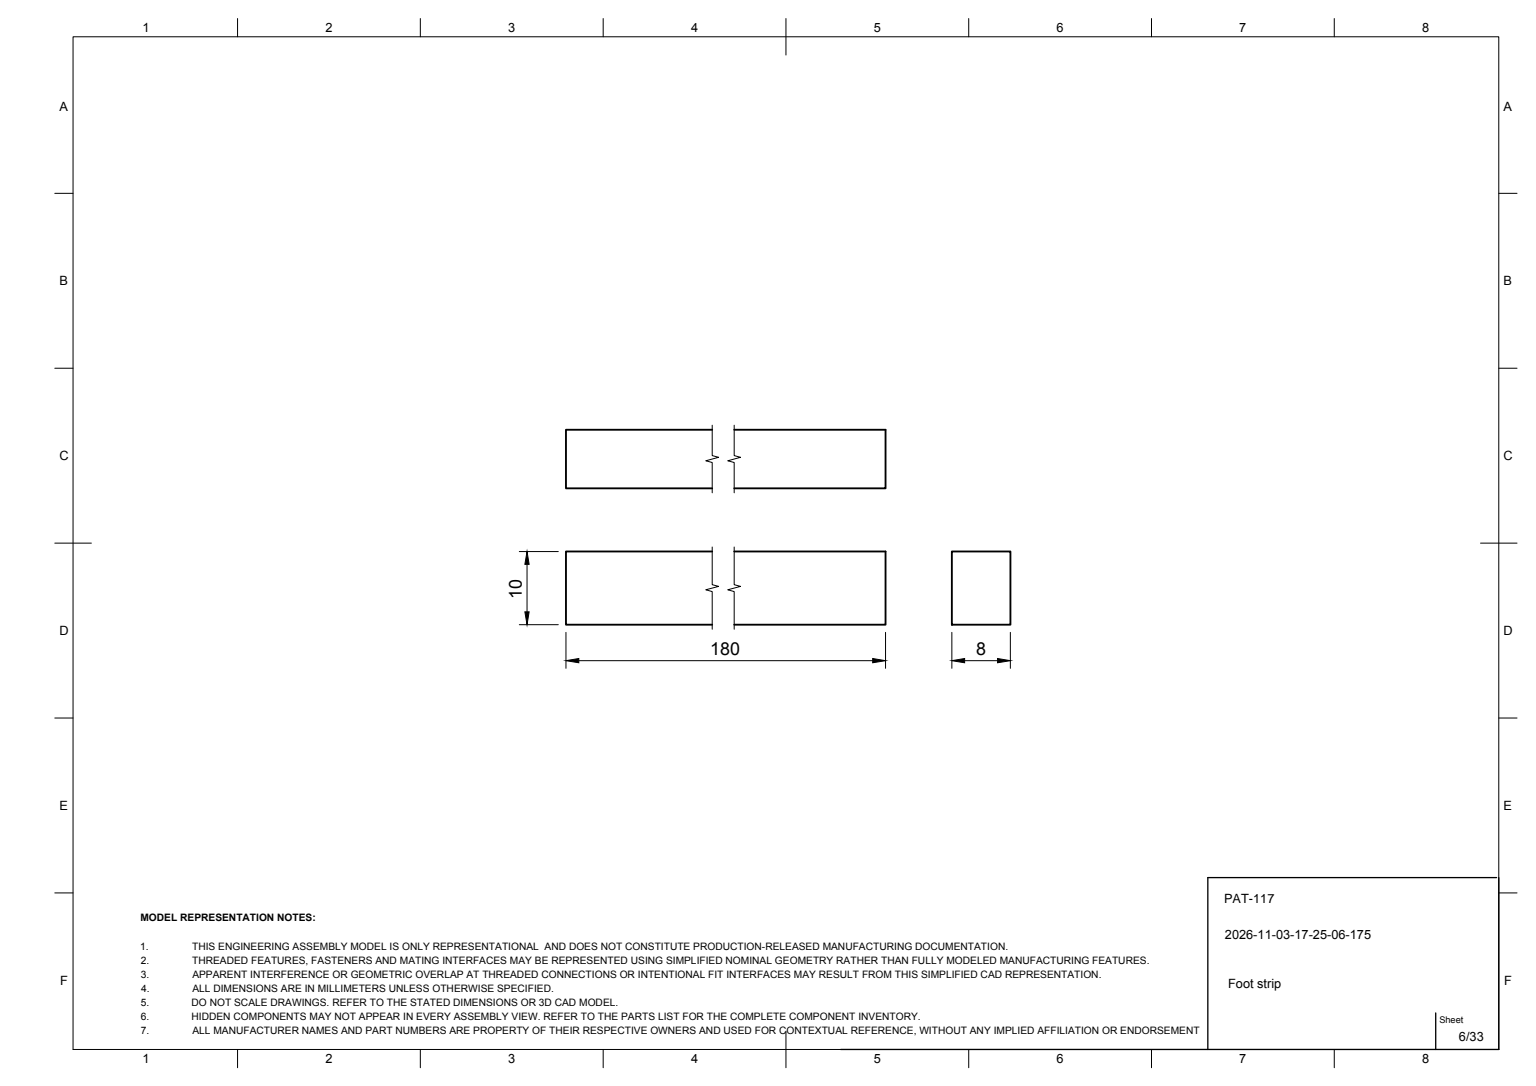
ISO-10303-21;
HEADER;
/* Generated by software containing ST-Developer
 * from STEP Tools, Inc. (www.steptools.com) 
 */

FILE_DESCRIPTION(
/* description */ ('Counterbalanced vertical column'),
/* implementation_level */ '2;1');

FILE_NAME(
/* name */ 'Foot strip.step',
/* time_stamp */ '2026-10-29T16:47:22-07:00',
/* author */ (''),
/* organization */ (''),
/* preprocessor_version */ 'ST-DEVELOPER v20.2',
/* originating_system */ 'Autodesk Translation Framework v15.17.0.0',
/* authorisation */ '');

FILE_SCHEMA (('AUTOMOTIVE_DESIGN { 1 0 10303 214 3 1 1 }'));
ENDSEC;

DATA;
#10=MECHANICAL_DESIGN_GEOMETRIC_PRESENTATION_REPRESENTATION('',(#351),#15040);
#281=SHAPE_REPRESENTATION_RELATIONSHIP('SRR','None',#15185,#316);
#316=ADVANCED_BREP_SHAPE_REPRESENTATION('',(#386),#15004);
#351=STYLED_ITEM('',(#15443),#386);
#386=MANIFOLD_SOLID_BREP('Body1',#7074);
#541=PLANE('',#7527);
#542=PLANE('',#7528);
#543=PLANE('',#7529);
#544=PLANE('',#7530);
#545=PLANE('',#7531);
#546=PLANE('',#7532);
#841=FACE_OUTER_BOUND('',#1252,.T.);
#842=FACE_OUTER_BOUND('',#1253,.T.);
#843=FACE_OUTER_BOUND('',#1254,.T.);
#844=FACE_OUTER_BOUND('',#1255,.T.);
#845=FACE_OUTER_BOUND('',#1256,.T.);
#846=FACE_OUTER_BOUND('',#1257,.T.);
#1252=EDGE_LOOP('',(#4842,#4843,#4844,#4845));
#1253=EDGE_LOOP('',(#4846,#4847,#4848,#4849));
#1254=EDGE_LOOP('',(#4850,#4851,#4852,#4853));
#1255=EDGE_LOOP('',(#4854,#4855,#4856,#4857));
#1256=EDGE_LOOP('',(#4858,#4859,#4860,#4861));
#1257=EDGE_LOOP('',(#4862,#4863,#4864,#4865));
#1768=LINE('',#10405,#2439);
#1769=LINE('',#10407,#2440);
#1770=LINE('',#10409,#2441);
#1771=LINE('',#10410,#2442);
#1772=LINE('',#10413,#2443);
#1773=LINE('',#10415,#2444);
#1774=LINE('',#10416,#2445);
#1775=LINE('',#10419,#2446);
#1776=LINE('',#10421,#2447);
#1777=LINE('',#10422,#2448);
#1778=LINE('',#10424,#2449);
#1779=LINE('',#10425,#2450);
#2439=VECTOR('',#8298,1.);
#2440=VECTOR('',#8299,1.);
#2441=VECTOR('',#8300,1.);
#2442=VECTOR('',#8301,1.);
#2443=VECTOR('',#8304,1.);
#2444=VECTOR('',#8305,1.);
#2445=VECTOR('',#8306,1.);
#2446=VECTOR('',#8309,1.);
#2447=VECTOR('',#8310,1.);
#2448=VECTOR('',#8311,1.);
#2449=VECTOR('',#8314,1.);
#2450=VECTOR('',#8315,1.);
#3324=VERTEX_POINT('',#10403);
#3325=VERTEX_POINT('',#10404);
#3326=VERTEX_POINT('',#10406);
#3327=VERTEX_POINT('',#10408);
#3328=VERTEX_POINT('',#10412);
#3329=VERTEX_POINT('',#10414);
#3330=VERTEX_POINT('',#10418);
#3331=VERTEX_POINT('',#10420);
#3922=EDGE_CURVE('',#3324,#3325,#1768,.T.);
#3923=EDGE_CURVE('',#3325,#3326,#1769,.T.);
#3924=EDGE_CURVE('',#3327,#3326,#1770,.T.);
#3925=EDGE_CURVE('',#3324,#3327,#1771,.T.);
#3926=EDGE_CURVE('',#3328,#3324,#1772,.T.);
#3927=EDGE_CURVE('',#3329,#3327,#1773,.T.);
#3928=EDGE_CURVE('',#3328,#3329,#1774,.T.);
#3929=EDGE_CURVE('',#3330,#3328,#1775,.T.);
#3930=EDGE_CURVE('',#3331,#3329,#1776,.T.);
#3931=EDGE_CURVE('',#3330,#3331,#1777,.T.);
#3932=EDGE_CURVE('',#3325,#3330,#1778,.T.);
#3933=EDGE_CURVE('',#3326,#3331,#1779,.T.);
#4842=ORIENTED_EDGE('',*,*,#3922,.T.);
#4843=ORIENTED_EDGE('',*,*,#3923,.T.);
#4844=ORIENTED_EDGE('',*,*,#3924,.F.);
#4845=ORIENTED_EDGE('',*,*,#3925,.F.);
#4846=ORIENTED_EDGE('',*,*,#3926,.T.);
#4847=ORIENTED_EDGE('',*,*,#3925,.T.);
#4848=ORIENTED_EDGE('',*,*,#3927,.F.);
#4849=ORIENTED_EDGE('',*,*,#3928,.F.);
#4850=ORIENTED_EDGE('',*,*,#3929,.T.);
#4851=ORIENTED_EDGE('',*,*,#3928,.T.);
#4852=ORIENTED_EDGE('',*,*,#3930,.F.);
#4853=ORIENTED_EDGE('',*,*,#3931,.F.);
#4854=ORIENTED_EDGE('',*,*,#3932,.T.);
#4855=ORIENTED_EDGE('',*,*,#3931,.T.);
#4856=ORIENTED_EDGE('',*,*,#3933,.F.);
#4857=ORIENTED_EDGE('',*,*,#3923,.F.);
#4858=ORIENTED_EDGE('',*,*,#3933,.T.);
#4859=ORIENTED_EDGE('',*,*,#3930,.T.);
#4860=ORIENTED_EDGE('',*,*,#3927,.T.);
#4861=ORIENTED_EDGE('',*,*,#3924,.T.);
#4862=ORIENTED_EDGE('',*,*,#3932,.F.);
#4863=ORIENTED_EDGE('',*,*,#3922,.F.);
#4864=ORIENTED_EDGE('',*,*,#3926,.F.);
#4865=ORIENTED_EDGE('',*,*,#3929,.F.);
#6683=ADVANCED_FACE('',(#841),#541,.T.);
#6684=ADVANCED_FACE('',(#842),#542,.T.);
#6685=ADVANCED_FACE('',(#843),#543,.T.);
#6686=ADVANCED_FACE('',(#844),#544,.T.);
#6687=ADVANCED_FACE('',(#845),#545,.T.);
#6688=ADVANCED_FACE('',(#846),#546,.F.);
#7074=CLOSED_SHELL('',(#6683,#6684,#6685,#6686,#6687,#6688));
#7526=AXIS2_PLACEMENT_3D('',#10401,#8294,#8295);
#7527=AXIS2_PLACEMENT_3D('',#10402,#8296,#8297);
#7528=AXIS2_PLACEMENT_3D('',#10411,#8302,#8303);
#7529=AXIS2_PLACEMENT_3D('',#10417,#8307,#8308);
#7530=AXIS2_PLACEMENT_3D('',#10423,#8312,#8313);
#7531=AXIS2_PLACEMENT_3D('',#10426,#8316,#8317);
#7532=AXIS2_PLACEMENT_3D('',#10427,#8318,#8319);
#8294=DIRECTION('axis',(0.,0.,1.));
#8295=DIRECTION('refdir',(1.,0.,0.));
#8296=DIRECTION('center_axis',(0.,1.,0.));
#8297=DIRECTION('ref_axis',(-1.,0.,0.));
#8298=DIRECTION('',(-1.,0.,0.));
#8299=DIRECTION('',(0.,0.,1.));
#8300=DIRECTION('',(-1.,0.,0.));
#8301=DIRECTION('',(0.,0.,1.));
#8302=DIRECTION('center_axis',(1.,0.,0.));
#8303=DIRECTION('ref_axis',(0.,1.,0.));
#8304=DIRECTION('',(0.,1.,0.));
#8305=DIRECTION('',(0.,1.,0.));
#8306=DIRECTION('',(0.,0.,1.));
#8307=DIRECTION('center_axis',(0.,-1.,0.));
#8308=DIRECTION('ref_axis',(1.,0.,0.));
#8309=DIRECTION('',(1.,0.,0.));
#8310=DIRECTION('',(1.,0.,0.));
#8311=DIRECTION('',(0.,0.,1.));
#8312=DIRECTION('center_axis',(-1.,0.,0.));
#8313=DIRECTION('ref_axis',(0.,-1.,0.));
#8314=DIRECTION('',(0.,-1.,0.));
#8315=DIRECTION('',(0.,-1.,0.));
#8316=DIRECTION('center_axis',(0.,0.,1.));
#8317=DIRECTION('ref_axis',(1.,0.,0.));
#8318=DIRECTION('center_axis',(0.,0.,1.));
#8319=DIRECTION('ref_axis',(1.,0.,0.));
#10401=CARTESIAN_POINT('',(0.,0.,0.));
#10402=CARTESIAN_POINT('Origin',(6.,-5.,-1.8));
#10403=CARTESIAN_POINT('',(6.,-5.,-1.8));
#10404=CARTESIAN_POINT('',(-12.,-5.,-1.8));
#10405=CARTESIAN_POINT('',(6.,-5.,-1.8));
#10406=CARTESIAN_POINT('',(-12.,-5.,-1.));
#10407=CARTESIAN_POINT('',(-12.,-5.,-1.8));
#10408=CARTESIAN_POINT('',(6.,-5.,-1.));
#10409=CARTESIAN_POINT('',(6.,-5.,-1.));
#10410=CARTESIAN_POINT('',(6.,-5.,-1.8));
#10411=CARTESIAN_POINT('Origin',(6.,-6.,-1.8));
#10412=CARTESIAN_POINT('',(6.,-6.,-1.8));
#10413=CARTESIAN_POINT('',(6.,-6.,-1.8));
#10414=CARTESIAN_POINT('',(6.,-6.,-1.));
#10415=CARTESIAN_POINT('',(6.,-6.,-1.));
#10416=CARTESIAN_POINT('',(6.,-6.,-1.8));
#10417=CARTESIAN_POINT('Origin',(-12.,-6.,-1.8));
#10418=CARTESIAN_POINT('',(-12.,-6.,-1.8));
#10419=CARTESIAN_POINT('',(-12.,-6.,-1.8));
#10420=CARTESIAN_POINT('',(-12.,-6.,-1.));
#10421=CARTESIAN_POINT('',(-12.,-6.,-1.));
#10422=CARTESIAN_POINT('',(-12.,-6.,-1.8));
#10423=CARTESIAN_POINT('Origin',(-12.,-5.,-1.8));
#10424=CARTESIAN_POINT('',(-12.,-5.,-1.8));
#10425=CARTESIAN_POINT('',(-12.,-5.,-1.));
#10426=CARTESIAN_POINT('Origin',(-3.,-5.5,-1.));
#10427=CARTESIAN_POINT('Origin',(-3.,-5.5,-1.8));
#14964=UNCERTAINTY_MEASURE_WITH_UNIT(LENGTH_MEASURE(0.001),#15041,
'DISTANCE_ACCURACY_VALUE',
'Maximum model space distance between geometric entities at asserted c
onnectivities');
#15000=UNCERTAINTY_MEASURE_WITH_UNIT(LENGTH_MEASURE(0.001),#15041,
'DISTANCE_ACCURACY_VALUE',
'Maximum model space distance between geometric entities at asserted c
onnectivities');
#15004=(
GEOMETRIC_REPRESENTATION_CONTEXT(3)
GLOBAL_UNCERTAINTY_ASSIGNED_CONTEXT((#14964))
GLOBAL_UNIT_ASSIGNED_CONTEXT((#15041,#15043,#15044))
REPRESENTATION_CONTEXT('','3D')
);
#15040=(
GEOMETRIC_REPRESENTATION_CONTEXT(3)
GLOBAL_UNCERTAINTY_ASSIGNED_CONTEXT((#15000))
GLOBAL_UNIT_ASSIGNED_CONTEXT((#15041,#15043,#15044))
REPRESENTATION_CONTEXT('','3D')
);
#15041=(
LENGTH_UNIT()
NAMED_UNIT(*)
SI_UNIT(.CENTI.,.METRE.)
);
#15043=(
NAMED_UNIT(*)
PLANE_ANGLE_UNIT()
SI_UNIT($,.RADIAN.)
);
#15044=(
NAMED_UNIT(*)
SI_UNIT($,.STERADIAN.)
SOLID_ANGLE_UNIT()
);
#15048=SHAPE_DEFINITION_REPRESENTATION(#15087,#15185);
#15087=PRODUCT_DEFINITION_SHAPE('',$,#15225);
#15185=SHAPE_REPRESENTATION('',(#7526),#15004);
#15221=PRODUCT_DEFINITION_CONTEXT('part definition',#15340,'design');
#15225=PRODUCT_DEFINITION('Foot strip','Foot strip',#15264,#15221);
#15264=PRODUCT_DEFINITION_FORMATION('',$,#15345);
#15340=APPLICATION_CONTEXT(
'Core Data for Automotive Mechanical Design Process');
#15341=PRODUCT_CONTEXT('part definition',#15340,'mechanical');
#15345=PRODUCT('Foot strip','Foot strip','Foot strip',(#15341));
#15437=COLOUR_RGB('Light Blue',0.38,0.62,0.78);
#15438=FILL_AREA_STYLE_COLOUR('',#15437);
#15439=FILL_AREA_STYLE('',(#15438));
#15440=SURFACE_STYLE_FILL_AREA(#15439);
#15441=SURFACE_SIDE_STYLE('',(#15440));
#15442=SURFACE_STYLE_USAGE(.BOTH.,#15441);
#15443=PRESENTATION_STYLE_ASSIGNMENT((#15442));
ENDSEC;
END-ISO-10303-21;
